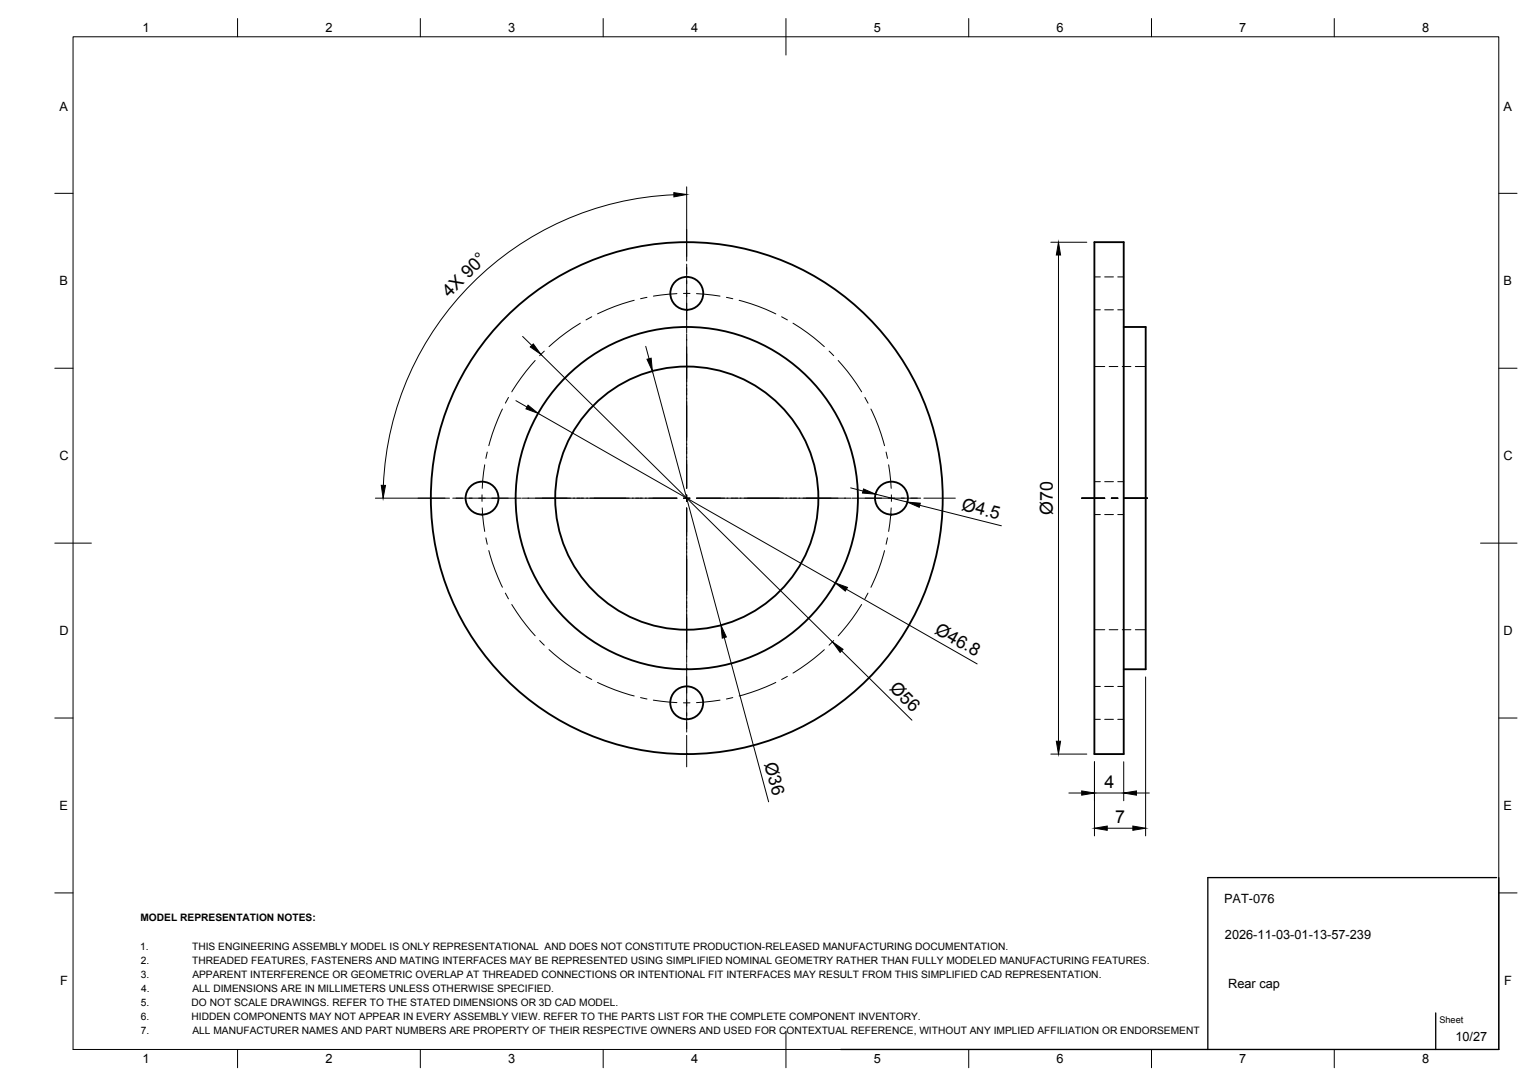
ISO-10303-21;
HEADER;
/* Generated by software containing ST-Developer
 * from STEP Tools, Inc. (www.steptools.com) 
 */

FILE_DESCRIPTION(
/* description */ ('Overhung pulley bearing cartridge'),
/* implementation_level */ '2;1');

FILE_NAME(
/* name */ 'Rear cap.step',
/* time_stamp */ '2026-10-28T03:22:33-07:00',
/* author */ (''),
/* organization */ (''),
/* preprocessor_version */ 'ST-DEVELOPER v20.2',
/* originating_system */ 'Autodesk Translation Framework v15.17.0.0',
/* authorisation */ '');

FILE_SCHEMA (('AUTOMOTIVE_DESIGN { 1 0 10303 214 3 1 1 }'));
ENDSEC;

DATA;
#10=MECHANICAL_DESIGN_GEOMETRIC_PRESENTATION_REPRESENTATION('',(#288),#10963);
#244=SHAPE_REPRESENTATION_RELATIONSHIP('SRR','None',#11064,#266);
#266=ADVANCED_BREP_SHAPE_REPRESENTATION('',(#318),#10944);
#288=STYLED_ITEM('',(#11246),#318);
#318=MANIFOLD_SOLID_BREP('Body1',#5655);
#385=FACE_BOUND('',#1028,.T.);
#386=FACE_BOUND('',#1032,.T.);
#387=FACE_BOUND('',#1033,.T.);
#388=FACE_BOUND('',#1034,.T.);
#389=FACE_BOUND('',#1035,.T.);
#390=FACE_BOUND('',#1036,.T.);
#391=FACE_BOUND('',#1038,.T.);
#392=FACE_BOUND('',#1039,.T.);
#393=FACE_BOUND('',#1040,.T.);
#394=FACE_BOUND('',#1041,.T.);
#395=FACE_BOUND('',#1042,.T.);
#476=PLANE('',#6088);
#477=PLANE('',#6095);
#478=PLANE('',#6096);
#649=FACE_OUTER_BOUND('',#1022,.T.);
#650=FACE_OUTER_BOUND('',#1023,.T.);
#651=FACE_OUTER_BOUND('',#1024,.T.);
#652=FACE_OUTER_BOUND('',#1025,.T.);
#653=FACE_OUTER_BOUND('',#1026,.T.);
#654=FACE_OUTER_BOUND('',#1027,.T.);
#655=FACE_OUTER_BOUND('',#1029,.T.);
#656=FACE_OUTER_BOUND('',#1030,.T.);
#657=FACE_OUTER_BOUND('',#1031,.T.);
#658=FACE_OUTER_BOUND('',#1037,.T.);
#1022=EDGE_LOOP('',(#3945,#3946,#3947,#3948));
#1023=EDGE_LOOP('',(#3949,#3950,#3951,#3952));
#1024=EDGE_LOOP('',(#3953,#3954,#3955,#3956));
#1025=EDGE_LOOP('',(#3957,#3958,#3959,#3960));
#1026=EDGE_LOOP('',(#3961,#3962,#3963,#3964));
#1027=EDGE_LOOP('',(#3965));
#1028=EDGE_LOOP('',(#3966));
#1029=EDGE_LOOP('',(#3967,#3968,#3969,#3970));
#1030=EDGE_LOOP('',(#3971,#3972,#3973,#3974));
#1031=EDGE_LOOP('',(#3975));
#1032=EDGE_LOOP('',(#3976));
#1033=EDGE_LOOP('',(#3977));
#1034=EDGE_LOOP('',(#3978));
#1035=EDGE_LOOP('',(#3979));
#1036=EDGE_LOOP('',(#3980));
#1037=EDGE_LOOP('',(#3981));
#1038=EDGE_LOOP('',(#3982));
#1039=EDGE_LOOP('',(#3983));
#1040=EDGE_LOOP('',(#3984));
#1041=EDGE_LOOP('',(#3985));
#1042=EDGE_LOOP('',(#3986));
#1406=LINE('',#8882,#1748);
#1407=LINE('',#8888,#1749);
#1408=LINE('',#8894,#1750);
#1409=LINE('',#8900,#1751);
#1410=LINE('',#8906,#1752);
#1411=LINE('',#8914,#1753);
#1412=LINE('',#8919,#1754);
#1748=VECTOR('',#7066,0.225);
#1749=VECTOR('',#7073,0.225);
#1750=VECTOR('',#7080,0.225);
#1751=VECTOR('',#7087,0.225);
#1752=VECTOR('',#7094,2.34);
#1753=VECTOR('',#7105,1.8);
#1754=VECTOR('',#7110,3.5);
#2080=CIRCLE('',#6074,0.225);
#2081=CIRCLE('',#6075,0.225);
#2082=CIRCLE('',#6077,0.225);
#2083=CIRCLE('',#6078,0.225);
#2084=CIRCLE('',#6080,0.225);
#2085=CIRCLE('',#6081,0.225);
#2086=CIRCLE('',#6083,0.225);
#2087=CIRCLE('',#6084,0.225);
#2088=CIRCLE('',#6086,2.34);
#2089=CIRCLE('',#6087,2.34);
#2090=CIRCLE('',#6089,1.8);
#2091=CIRCLE('',#6091,1.8);
#2092=CIRCLE('',#6093,3.5);
#2093=CIRCLE('',#6094,3.5);
#2479=VERTEX_POINT('',#8879);
#2480=VERTEX_POINT('',#8881);
#2481=VERTEX_POINT('',#8885);
#2482=VERTEX_POINT('',#8887);
#2483=VERTEX_POINT('',#8891);
#2484=VERTEX_POINT('',#8893);
#2485=VERTEX_POINT('',#8897);
#2486=VERTEX_POINT('',#8899);
#2487=VERTEX_POINT('',#8903);
#2488=VERTEX_POINT('',#8905);
#2489=VERTEX_POINT('',#8909);
#2490=VERTEX_POINT('',#8912);
#2491=VERTEX_POINT('',#8916);
#2492=VERTEX_POINT('',#8918);
#3042=EDGE_CURVE('',#2479,#2479,#2080,.T.);
#3043=EDGE_CURVE('',#2479,#2480,#1406,.T.);
#3044=EDGE_CURVE('',#2480,#2480,#2081,.T.);
#3045=EDGE_CURVE('',#2481,#2481,#2082,.T.);
#3046=EDGE_CURVE('',#2481,#2482,#1407,.T.);
#3047=EDGE_CURVE('',#2482,#2482,#2083,.T.);
#3048=EDGE_CURVE('',#2483,#2483,#2084,.T.);
#3049=EDGE_CURVE('',#2483,#2484,#1408,.T.);
#3050=EDGE_CURVE('',#2484,#2484,#2085,.T.);
#3051=EDGE_CURVE('',#2485,#2485,#2086,.T.);
#3052=EDGE_CURVE('',#2485,#2486,#1409,.T.);
#3053=EDGE_CURVE('',#2486,#2486,#2087,.T.);
#3054=EDGE_CURVE('',#2487,#2487,#2088,.T.);
#3055=EDGE_CURVE('',#2487,#2488,#1410,.T.);
#3056=EDGE_CURVE('',#2488,#2488,#2089,.T.);
#3057=EDGE_CURVE('',#2489,#2489,#2090,.T.);
#3058=EDGE_CURVE('',#2490,#2490,#2091,.T.);
#3059=EDGE_CURVE('',#2490,#2489,#1411,.T.);
#3060=EDGE_CURVE('',#2491,#2491,#2092,.T.);
#3061=EDGE_CURVE('',#2491,#2492,#1412,.T.);
#3062=EDGE_CURVE('',#2492,#2492,#2093,.T.);
#3945=ORIENTED_EDGE('',*,*,#3042,.F.);
#3946=ORIENTED_EDGE('',*,*,#3043,.T.);
#3947=ORIENTED_EDGE('',*,*,#3044,.F.);
#3948=ORIENTED_EDGE('',*,*,#3043,.F.);
#3949=ORIENTED_EDGE('',*,*,#3045,.F.);
#3950=ORIENTED_EDGE('',*,*,#3046,.T.);
#3951=ORIENTED_EDGE('',*,*,#3047,.F.);
#3952=ORIENTED_EDGE('',*,*,#3046,.F.);
#3953=ORIENTED_EDGE('',*,*,#3048,.F.);
#3954=ORIENTED_EDGE('',*,*,#3049,.T.);
#3955=ORIENTED_EDGE('',*,*,#3050,.F.);
#3956=ORIENTED_EDGE('',*,*,#3049,.F.);
#3957=ORIENTED_EDGE('',*,*,#3051,.F.);
#3958=ORIENTED_EDGE('',*,*,#3052,.T.);
#3959=ORIENTED_EDGE('',*,*,#3053,.F.);
#3960=ORIENTED_EDGE('',*,*,#3052,.F.);
#3961=ORIENTED_EDGE('',*,*,#3054,.F.);
#3962=ORIENTED_EDGE('',*,*,#3055,.T.);
#3963=ORIENTED_EDGE('',*,*,#3056,.T.);
#3964=ORIENTED_EDGE('',*,*,#3055,.F.);
#3965=ORIENTED_EDGE('',*,*,#3056,.F.);
#3966=ORIENTED_EDGE('',*,*,#3057,.F.);
#3967=ORIENTED_EDGE('',*,*,#3058,.F.);
#3968=ORIENTED_EDGE('',*,*,#3059,.T.);
#3969=ORIENTED_EDGE('',*,*,#3057,.T.);
#3970=ORIENTED_EDGE('',*,*,#3059,.F.);
#3971=ORIENTED_EDGE('',*,*,#3060,.F.);
#3972=ORIENTED_EDGE('',*,*,#3061,.T.);
#3973=ORIENTED_EDGE('',*,*,#3062,.T.);
#3974=ORIENTED_EDGE('',*,*,#3061,.F.);
#3975=ORIENTED_EDGE('',*,*,#3060,.T.);
#3976=ORIENTED_EDGE('',*,*,#3058,.T.);
#3977=ORIENTED_EDGE('',*,*,#3053,.T.);
#3978=ORIENTED_EDGE('',*,*,#3050,.T.);
#3979=ORIENTED_EDGE('',*,*,#3047,.T.);
#3980=ORIENTED_EDGE('',*,*,#3044,.T.);
#3981=ORIENTED_EDGE('',*,*,#3062,.F.);
#3982=ORIENTED_EDGE('',*,*,#3054,.T.);
#3983=ORIENTED_EDGE('',*,*,#3051,.T.);
#3984=ORIENTED_EDGE('',*,*,#3048,.T.);
#3985=ORIENTED_EDGE('',*,*,#3045,.T.);
#3986=ORIENTED_EDGE('',*,*,#3042,.T.);
#5197=CYLINDRICAL_SURFACE('',#6073,0.225);
#5198=CYLINDRICAL_SURFACE('',#6076,0.225);
#5199=CYLINDRICAL_SURFACE('',#6079,0.225);
#5200=CYLINDRICAL_SURFACE('',#6082,0.225);
#5201=CYLINDRICAL_SURFACE('',#6085,2.34);
#5202=CYLINDRICAL_SURFACE('',#6090,1.8);
#5203=CYLINDRICAL_SURFACE('',#6092,3.5);
#5393=ADVANCED_FACE('',(#649),#5197,.F.);
#5394=ADVANCED_FACE('',(#650),#5198,.F.);
#5395=ADVANCED_FACE('',(#651),#5199,.F.);
#5396=ADVANCED_FACE('',(#652),#5200,.F.);
#5397=ADVANCED_FACE('',(#653),#5201,.T.);
#5398=ADVANCED_FACE('',(#654,#385),#476,.F.);
#5399=ADVANCED_FACE('',(#655),#5202,.F.);
#5400=ADVANCED_FACE('',(#656),#5203,.T.);
#5401=ADVANCED_FACE('',(#657,#386,#387,#388,#389,#390),#477,.T.);
#5402=ADVANCED_FACE('',(#658,#391,#392,#393,#394,#395),#478,.F.);
#5655=CLOSED_SHELL('',(#5393,#5394,#5395,#5396,#5397,#5398,#5399,#5400,
#5401,#5402));
#6072=AXIS2_PLACEMENT_3D('',#8877,#7060,#7061);
#6073=AXIS2_PLACEMENT_3D('',#8878,#7062,#7063);
#6074=AXIS2_PLACEMENT_3D('',#8880,#7064,#7065);
#6075=AXIS2_PLACEMENT_3D('',#8883,#7067,#7068);
#6076=AXIS2_PLACEMENT_3D('',#8884,#7069,#7070);
#6077=AXIS2_PLACEMENT_3D('',#8886,#7071,#7072);
#6078=AXIS2_PLACEMENT_3D('',#8889,#7074,#7075);
#6079=AXIS2_PLACEMENT_3D('',#8890,#7076,#7077);
#6080=AXIS2_PLACEMENT_3D('',#8892,#7078,#7079);
#6081=AXIS2_PLACEMENT_3D('',#8895,#7081,#7082);
#6082=AXIS2_PLACEMENT_3D('',#8896,#7083,#7084);
#6083=AXIS2_PLACEMENT_3D('',#8898,#7085,#7086);
#6084=AXIS2_PLACEMENT_3D('',#8901,#7088,#7089);
#6085=AXIS2_PLACEMENT_3D('',#8902,#7090,#7091);
#6086=AXIS2_PLACEMENT_3D('',#8904,#7092,#7093);
#6087=AXIS2_PLACEMENT_3D('',#8907,#7095,#7096);
#6088=AXIS2_PLACEMENT_3D('',#8908,#7097,#7098);
#6089=AXIS2_PLACEMENT_3D('',#8910,#7099,#7100);
#6090=AXIS2_PLACEMENT_3D('',#8911,#7101,#7102);
#6091=AXIS2_PLACEMENT_3D('',#8913,#7103,#7104);
#6092=AXIS2_PLACEMENT_3D('',#8915,#7106,#7107);
#6093=AXIS2_PLACEMENT_3D('',#8917,#7108,#7109);
#6094=AXIS2_PLACEMENT_3D('',#8920,#7111,#7112);
#6095=AXIS2_PLACEMENT_3D('',#8921,#7113,#7114);
#6096=AXIS2_PLACEMENT_3D('',#8922,#7115,#7116);
#7060=DIRECTION('axis',(0.,0.,1.));
#7061=DIRECTION('refdir',(1.,0.,0.));
#7062=DIRECTION('center_axis',(0.,1.,0.));
#7063=DIRECTION('ref_axis',(1.,0.,0.));
#7064=DIRECTION('center_axis',(0.,1.,0.));
#7065=DIRECTION('ref_axis',(1.,0.,0.));
#7066=DIRECTION('',(0.,1.,0.));
#7067=DIRECTION('center_axis',(0.,-1.,0.));
#7068=DIRECTION('ref_axis',(1.,0.,0.));
#7069=DIRECTION('center_axis',(0.,1.,0.));
#7070=DIRECTION('ref_axis',(1.,0.,0.));
#7071=DIRECTION('center_axis',(0.,1.,0.));
#7072=DIRECTION('ref_axis',(1.,0.,0.));
#7073=DIRECTION('',(0.,1.,0.));
#7074=DIRECTION('center_axis',(0.,-1.,0.));
#7075=DIRECTION('ref_axis',(1.,0.,0.));
#7076=DIRECTION('center_axis',(0.,1.,0.));
#7077=DIRECTION('ref_axis',(1.,0.,0.));
#7078=DIRECTION('center_axis',(0.,1.,0.));
#7079=DIRECTION('ref_axis',(1.,0.,0.));
#7080=DIRECTION('',(0.,1.,0.));
#7081=DIRECTION('center_axis',(0.,-1.,0.));
#7082=DIRECTION('ref_axis',(1.,0.,0.));
#7083=DIRECTION('center_axis',(0.,1.,0.));
#7084=DIRECTION('ref_axis',(1.,0.,0.));
#7085=DIRECTION('center_axis',(0.,1.,0.));
#7086=DIRECTION('ref_axis',(1.,0.,0.));
#7087=DIRECTION('',(0.,1.,0.));
#7088=DIRECTION('center_axis',(0.,-1.,0.));
#7089=DIRECTION('ref_axis',(1.,0.,0.));
#7090=DIRECTION('center_axis',(0.,1.,0.));
#7091=DIRECTION('ref_axis',(1.,0.,0.));
#7092=DIRECTION('center_axis',(0.,1.,0.));
#7093=DIRECTION('ref_axis',(1.,0.,0.));
#7094=DIRECTION('',(0.,-1.,0.));
#7095=DIRECTION('center_axis',(0.,1.,0.));
#7096=DIRECTION('ref_axis',(1.,0.,0.));
#7097=DIRECTION('center_axis',(0.,1.,0.));
#7098=DIRECTION('ref_axis',(1.,0.,0.));
#7099=DIRECTION('center_axis',(0.,-1.,0.));
#7100=DIRECTION('ref_axis',(1.,0.,0.));
#7101=DIRECTION('center_axis',(0.,1.,0.));
#7102=DIRECTION('ref_axis',(1.,0.,0.));
#7103=DIRECTION('center_axis',(0.,-1.,0.));
#7104=DIRECTION('ref_axis',(1.,0.,0.));
#7105=DIRECTION('',(0.,-1.,0.));
#7106=DIRECTION('center_axis',(0.,1.,0.));
#7107=DIRECTION('ref_axis',(1.,0.,0.));
#7108=DIRECTION('center_axis',(0.,1.,0.));
#7109=DIRECTION('ref_axis',(1.,0.,0.));
#7110=DIRECTION('',(0.,-1.,0.));
#7111=DIRECTION('center_axis',(0.,1.,0.));
#7112=DIRECTION('ref_axis',(1.,0.,0.));
#7113=DIRECTION('center_axis',(0.,1.,0.));
#7114=DIRECTION('ref_axis',(1.,0.,0.));
#7115=DIRECTION('center_axis',(0.,1.,0.));
#7116=DIRECTION('ref_axis',(1.,0.,0.));
#8877=CARTESIAN_POINT('',(0.,0.,0.));
#8878=CARTESIAN_POINT('Origin',(-2.8,5.9,4.5));
#8879=CARTESIAN_POINT('',(-3.025,6.,4.5));
#8880=CARTESIAN_POINT('Origin',(-2.8,6.,4.5));
#8881=CARTESIAN_POINT('',(-3.025,6.4,4.5));
#8882=CARTESIAN_POINT('',(-3.025,5.9,4.5));
#8883=CARTESIAN_POINT('Origin',(-2.8,6.4,4.5));
#8884=CARTESIAN_POINT('Origin',(1.71450551880629E-16,5.9,7.3));
#8885=CARTESIAN_POINT('',(-0.225,6.,7.3));
#8886=CARTESIAN_POINT('Origin',(1.71450551880629E-16,6.,7.3));
#8887=CARTESIAN_POINT('',(-0.225,6.4,7.3));
#8888=CARTESIAN_POINT('',(-0.225,5.9,7.3));
#8889=CARTESIAN_POINT('Origin',(1.71450551880629E-16,6.4,7.3));
#8890=CARTESIAN_POINT('Origin',(2.8,5.9,4.5));
#8891=CARTESIAN_POINT('',(2.575,6.,4.5));
#8892=CARTESIAN_POINT('Origin',(2.8,6.,4.5));
#8893=CARTESIAN_POINT('',(2.575,6.4,4.5));
#8894=CARTESIAN_POINT('',(2.575,5.9,4.5));
#8895=CARTESIAN_POINT('Origin',(2.8,6.4,4.5));
#8896=CARTESIAN_POINT('Origin',(-5.14351655641888E-16,5.9,1.7));
#8897=CARTESIAN_POINT('',(-0.225000000000001,6.,1.7));
#8898=CARTESIAN_POINT('Origin',(-5.14351655641888E-16,6.,1.7));
#8899=CARTESIAN_POINT('',(-0.225000000000001,6.4,1.7));
#8900=CARTESIAN_POINT('',(-0.225000000000001,5.9,1.7));
#8901=CARTESIAN_POINT('Origin',(-5.14351655641888E-16,6.4,1.7));
#8902=CARTESIAN_POINT('Origin',(0.,5.7,4.5));
#8903=CARTESIAN_POINT('',(-2.34,6.,4.5));
#8904=CARTESIAN_POINT('Origin',(0.,6.,4.5));
#8905=CARTESIAN_POINT('',(-2.34,5.7,4.5));
#8906=CARTESIAN_POINT('',(-2.34,5.7,4.5));
#8907=CARTESIAN_POINT('Origin',(0.,5.7,4.5));
#8908=CARTESIAN_POINT('Origin',(0.,5.7,4.5));
#8909=CARTESIAN_POINT('',(-1.8,5.7,4.5));
#8910=CARTESIAN_POINT('Origin',(0.,5.7,4.5));
#8911=CARTESIAN_POINT('Origin',(0.,6.,4.5));
#8912=CARTESIAN_POINT('',(-1.8,6.4,4.5));
#8913=CARTESIAN_POINT('Origin',(0.,6.4,4.5));
#8914=CARTESIAN_POINT('',(-1.8,6.,4.5));
#8915=CARTESIAN_POINT('Origin',(0.,6.,4.5));
#8916=CARTESIAN_POINT('',(-3.5,6.4,4.5));
#8917=CARTESIAN_POINT('Origin',(0.,6.4,4.5));
#8918=CARTESIAN_POINT('',(-3.5,6.,4.5));
#8919=CARTESIAN_POINT('',(-3.5,6.,4.5));
#8920=CARTESIAN_POINT('Origin',(0.,6.,4.5));
#8921=CARTESIAN_POINT('Origin',(0.,6.4,4.5));
#8922=CARTESIAN_POINT('Origin',(0.,6.,4.5));
#10917=UNCERTAINTY_MEASURE_WITH_UNIT(LENGTH_MEASURE(0.001),#10964,
'DISTANCE_ACCURACY_VALUE',
'Maximum model space distance between geometric entities at asserted c
onnectivities');
#10936=UNCERTAINTY_MEASURE_WITH_UNIT(LENGTH_MEASURE(0.001),#10964,
'DISTANCE_ACCURACY_VALUE',
'Maximum model space distance between geometric entities at asserted c
onnectivities');
#10944=(
GEOMETRIC_REPRESENTATION_CONTEXT(3)
GLOBAL_UNCERTAINTY_ASSIGNED_CONTEXT((#10917))
GLOBAL_UNIT_ASSIGNED_CONTEXT((#10964,#10966,#10967))
REPRESENTATION_CONTEXT('','3D')
);
#10963=(
GEOMETRIC_REPRESENTATION_CONTEXT(3)
GLOBAL_UNCERTAINTY_ASSIGNED_CONTEXT((#10936))
GLOBAL_UNIT_ASSIGNED_CONTEXT((#10964,#10966,#10967))
REPRESENTATION_CONTEXT('','3D')
);
#10964=(
LENGTH_UNIT()
NAMED_UNIT(*)
SI_UNIT(.CENTI.,.METRE.)
);
#10966=(
NAMED_UNIT(*)
PLANE_ANGLE_UNIT()
SI_UNIT($,.RADIAN.)
);
#10967=(
NAMED_UNIT(*)
SI_UNIT($,.STERADIAN.)
SOLID_ANGLE_UNIT()
);
#10975=SHAPE_DEFINITION_REPRESENTATION(#11001,#11064);
#11001=PRODUCT_DEFINITION_SHAPE('',$,#11091);
#11064=SHAPE_REPRESENTATION('',(#6072),#10944);
#11083=PRODUCT_DEFINITION_CONTEXT('part definition',#11163,'design');
#11091=PRODUCT_DEFINITION('Rear cap','Rear cap',#11117,#11083);
#11117=PRODUCT_DEFINITION_FORMATION('',$,#11172);
#11163=APPLICATION_CONTEXT(
'Core Data for Automotive Mechanical Design Process');
#11164=PRODUCT_CONTEXT('part definition',#11163,'mechanical');
#11172=PRODUCT('Rear cap','Rear cap','Rear cap',(#11164));
#11240=COLOUR_RGB('Sky Blue',0.24,0.69,0.87);
#11241=FILL_AREA_STYLE_COLOUR('',#11240);
#11242=FILL_AREA_STYLE('',(#11241));
#11243=SURFACE_STYLE_FILL_AREA(#11242);
#11244=SURFACE_SIDE_STYLE('',(#11243));
#11245=SURFACE_STYLE_USAGE(.BOTH.,#11244);
#11246=PRESENTATION_STYLE_ASSIGNMENT((#11245));
ENDSEC;
END-ISO-10303-21;
